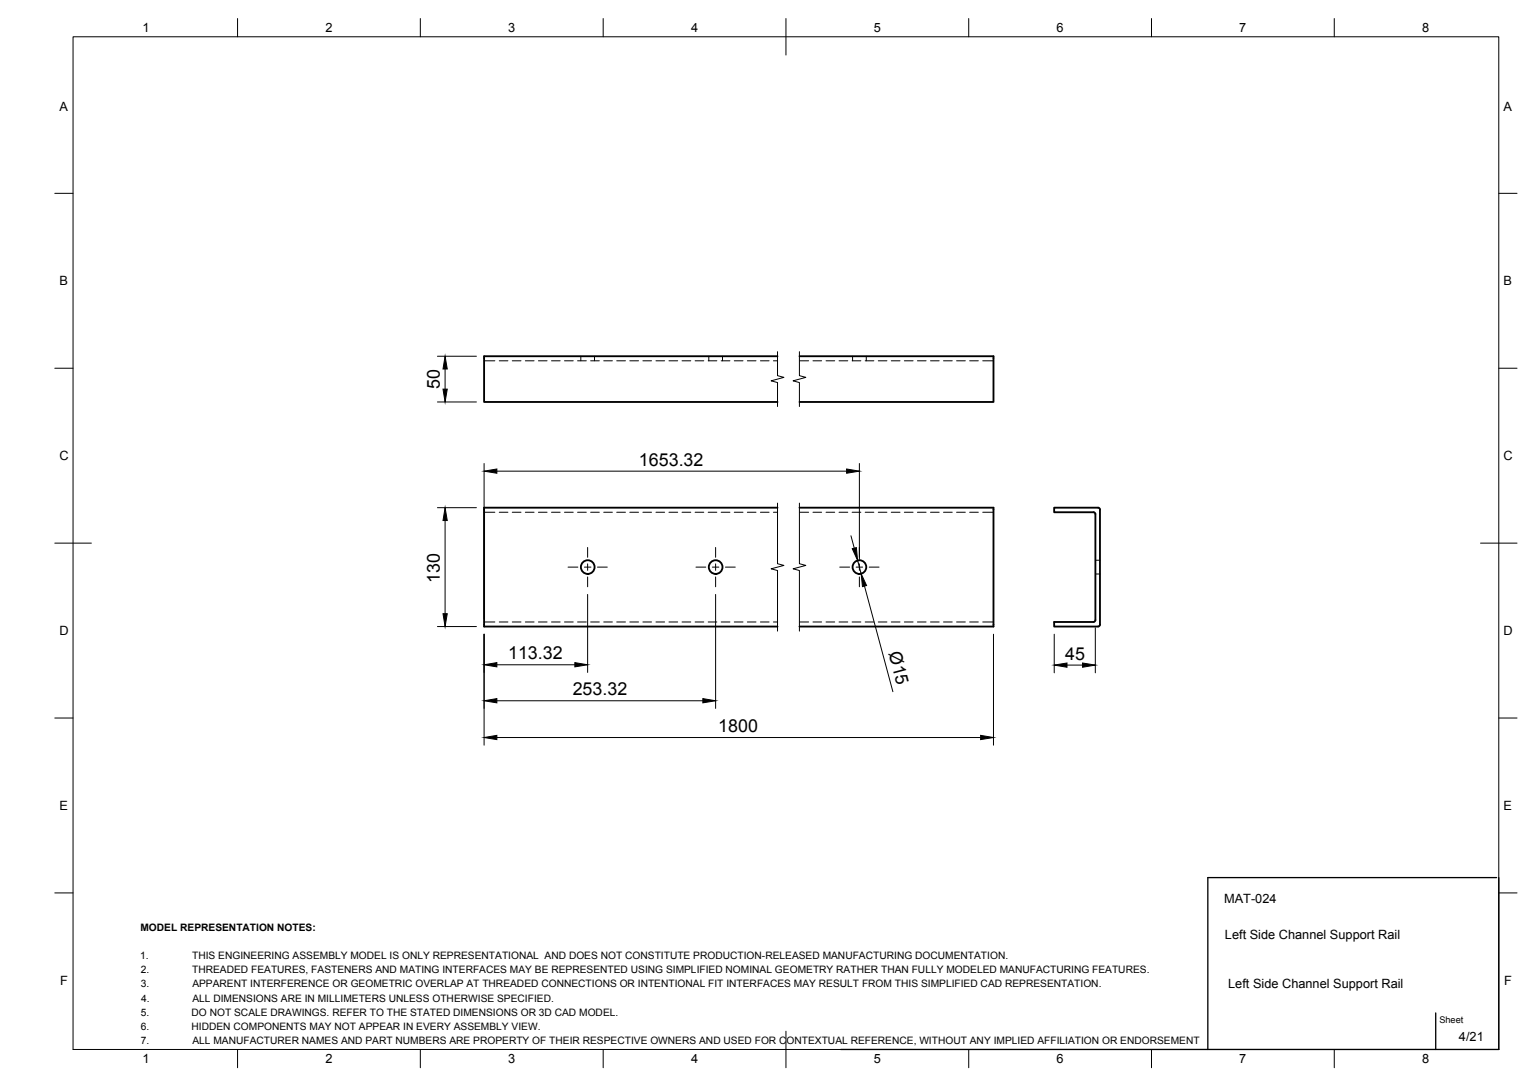
ISO-10303-21;
HEADER;
/* Generated by software containing ST-Developer
 * from STEP Tools, Inc. (www.steptools.com) 
 */

FILE_DESCRIPTION(
/* description */ ('STEP AP214'),
/* implementation_level */ '2;1');

FILE_NAME(
/* name */ 'Left Side Channel Support Rail.step',
/* time_stamp */ '2026-11-14T06:34:07-08:00',
/* author */ (''),
/* organization */ (''),
/* preprocessor_version */ 'ST-DEVELOPER v20.2',
/* originating_system */ 'Autodesk Translation Framework v15.17.0.0',
/* authorisation */ '');

FILE_SCHEMA (('AUTOMOTIVE_DESIGN { 1 0 10303 214 3 1 1 }'));
ENDSEC;

DATA;
#10=MECHANICAL_DESIGN_GEOMETRIC_PRESENTATION_REPRESENTATION('',(#7257),#310623);
#7223=SHAPE_REPRESENTATION_RELATIONSHIP('SRR','None',#310895,#7240);
#7240=ADVANCED_BREP_SHAPE_REPRESENTATION('',(#7325),#310604);
#7257=STYLED_ITEM('',(#311004),#7325);
#7325=MANIFOLD_SOLID_BREP('Body1',#93707);
#7415=FACE_BOUND('',#14492,.T.);
#7416=FACE_BOUND('',#14493,.T.);
#7417=FACE_BOUND('',#14494,.T.);
#7418=FACE_BOUND('',#14495,.T.);
#7419=FACE_BOUND('',#14496,.T.);
#7420=FACE_BOUND('',#14497,.T.);
#7421=FACE_BOUND('',#14498,.T.);
#7422=FACE_BOUND('',#14499,.T.);
#7423=FACE_BOUND('',#14500,.T.);
#7424=FACE_BOUND('',#14501,.T.);
#7425=FACE_BOUND('',#14502,.T.);
#7426=FACE_BOUND('',#14503,.T.);
#7427=FACE_BOUND('',#14508,.T.);
#7428=FACE_BOUND('',#14509,.T.);
#7429=FACE_BOUND('',#14510,.T.);
#7430=FACE_BOUND('',#14511,.T.);
#7431=FACE_BOUND('',#14512,.T.);
#7432=FACE_BOUND('',#14513,.T.);
#7433=FACE_BOUND('',#14514,.T.);
#7434=FACE_BOUND('',#14515,.T.);
#7435=FACE_BOUND('',#14516,.T.);
#7436=FACE_BOUND('',#14517,.T.);
#7437=FACE_BOUND('',#14518,.T.);
#7438=FACE_BOUND('',#14519,.T.);
#7716=PLANE('',#94060);
#7717=PLANE('',#94061);
#7718=PLANE('',#94062);
#7719=PLANE('',#94063);
#7720=PLANE('',#94064);
#7721=PLANE('',#94065);
#7722=PLANE('',#94066);
#7723=PLANE('',#94067);
#7724=PLANE('',#94068);
#7725=PLANE('',#94073);
#8714=FACE_OUTER_BOUND('',#14477,.T.);
#8715=FACE_OUTER_BOUND('',#14478,.T.);
#8716=FACE_OUTER_BOUND('',#14479,.T.);
#8717=FACE_OUTER_BOUND('',#14480,.T.);
#8718=FACE_OUTER_BOUND('',#14481,.T.);
#8719=FACE_OUTER_BOUND('',#14482,.T.);
#8720=FACE_OUTER_BOUND('',#14483,.T.);
#8721=FACE_OUTER_BOUND('',#14484,.T.);
#8722=FACE_OUTER_BOUND('',#14485,.T.);
#8723=FACE_OUTER_BOUND('',#14486,.T.);
#8724=FACE_OUTER_BOUND('',#14487,.T.);
#8725=FACE_OUTER_BOUND('',#14488,.T.);
#8726=FACE_OUTER_BOUND('',#14489,.T.);
#8727=FACE_OUTER_BOUND('',#14490,.T.);
#8728=FACE_OUTER_BOUND('',#14491,.T.);
#8729=FACE_OUTER_BOUND('',#14504,.T.);
#8730=FACE_OUTER_BOUND('',#14505,.T.);
#8731=FACE_OUTER_BOUND('',#14506,.T.);
#8732=FACE_OUTER_BOUND('',#14507,.T.);
#8733=FACE_OUTER_BOUND('',#14520,.T.);
#8734=FACE_OUTER_BOUND('',#14521,.T.);
#8735=FACE_OUTER_BOUND('',#14522,.T.);
#8736=FACE_OUTER_BOUND('',#14523,.T.);
#8737=FACE_OUTER_BOUND('',#14524,.T.);
#8738=FACE_OUTER_BOUND('',#14525,.T.);
#8739=FACE_OUTER_BOUND('',#14526,.T.);
#14477=EDGE_LOOP('',(#57801,#57802,#57803,#57804));
#14478=EDGE_LOOP('',(#57805,#57806,#57807,#57808));
#14479=EDGE_LOOP('',(#57809,#57810,#57811,#57812));
#14480=EDGE_LOOP('',(#57813,#57814,#57815,#57816));
#14481=EDGE_LOOP('',(#57817,#57818,#57819,#57820));
#14482=EDGE_LOOP('',(#57821,#57822,#57823,#57824));
#14483=EDGE_LOOP('',(#57825,#57826,#57827,#57828));
#14484=EDGE_LOOP('',(#57829,#57830,#57831,#57832));
#14485=EDGE_LOOP('',(#57833,#57834,#57835,#57836));
#14486=EDGE_LOOP('',(#57837,#57838,#57839,#57840));
#14487=EDGE_LOOP('',(#57841,#57842,#57843,#57844));
#14488=EDGE_LOOP('',(#57845,#57846,#57847,#57848));
#14489=EDGE_LOOP('',(#57849,#57850,#57851,#57852));
#14490=EDGE_LOOP('',(#57853,#57854,#57855,#57856));
#14491=EDGE_LOOP('',(#57857,#57858,#57859,#57860));
#14492=EDGE_LOOP('',(#57861));
#14493=EDGE_LOOP('',(#57862));
#14494=EDGE_LOOP('',(#57863));
#14495=EDGE_LOOP('',(#57864));
#14496=EDGE_LOOP('',(#57865));
#14497=EDGE_LOOP('',(#57866));
#14498=EDGE_LOOP('',(#57867));
#14499=EDGE_LOOP('',(#57868));
#14500=EDGE_LOOP('',(#57869));
#14501=EDGE_LOOP('',(#57870));
#14502=EDGE_LOOP('',(#57871));
#14503=EDGE_LOOP('',(#57872));
#14504=EDGE_LOOP('',(#57873,#57874,#57875,#57876));
#14505=EDGE_LOOP('',(#57877,#57878,#57879,#57880));
#14506=EDGE_LOOP('',(#57881,#57882,#57883,#57884));
#14507=EDGE_LOOP('',(#57885,#57886,#57887,#57888));
#14508=EDGE_LOOP('',(#57889));
#14509=EDGE_LOOP('',(#57890));
#14510=EDGE_LOOP('',(#57891));
#14511=EDGE_LOOP('',(#57892));
#14512=EDGE_LOOP('',(#57893));
#14513=EDGE_LOOP('',(#57894));
#14514=EDGE_LOOP('',(#57895));
#14515=EDGE_LOOP('',(#57896));
#14516=EDGE_LOOP('',(#57897));
#14517=EDGE_LOOP('',(#57898));
#14518=EDGE_LOOP('',(#57899));
#14519=EDGE_LOOP('',(#57900));
#14520=EDGE_LOOP('',(#57901,#57902,#57903,#57904));
#14521=EDGE_LOOP('',(#57905,#57906,#57907,#57908,#57909,#57910,#57911,#57912,
#57913,#57914,#57915,#57916));
#14522=EDGE_LOOP('',(#57917,#57918,#57919,#57920,#57921,#57922,#57923,#57924,
#57925,#57926,#57927,#57928));
#14523=EDGE_LOOP('',(#57929,#57930,#57931,#57932));
#14524=EDGE_LOOP('',(#57933,#57934,#57935,#57936));
#14525=EDGE_LOOP('',(#57937,#57938,#57939,#57940));
#14526=EDGE_LOOP('',(#57941,#57942,#57943,#57944));
#20521=LINE('',#131166,#24868);
#20522=LINE('',#131172,#24869);
#20523=LINE('',#131178,#24870);
#20524=LINE('',#131184,#24871);
#20525=LINE('',#131190,#24872);
#20526=LINE('',#131196,#24873);
#20527=LINE('',#131202,#24874);
#20528=LINE('',#131208,#24875);
#20529=LINE('',#131214,#24876);
#20530=LINE('',#131220,#24877);
#20531=LINE('',#131226,#24878);
#20532=LINE('',#131232,#24879);
#20533=LINE('',#131237,#24880);
#20534=LINE('',#131239,#24881);
#20535=LINE('',#131241,#24882);
#20536=LINE('',#131242,#24883);
#20537=LINE('',#131245,#24884);
#20538=LINE('',#131247,#24885);
#20539=LINE('',#131248,#24886);
#20540=LINE('',#131252,#24887);
#20541=LINE('',#131254,#24888);
#20542=LINE('',#131256,#24889);
#20543=LINE('',#131257,#24890);
#20544=LINE('',#131261,#24891);
#20545=LINE('',#131263,#24892);
#20546=LINE('',#131265,#24893);
#20547=LINE('',#131266,#24894);
#20548=LINE('',#131269,#24895);
#20549=LINE('',#131271,#24896);
#20550=LINE('',#131272,#24897);
#20551=LINE('',#131275,#24898);
#20552=LINE('',#131277,#24899);
#20553=LINE('',#131278,#24900);
#20554=LINE('',#131282,#24901);
#20555=LINE('',#131284,#24902);
#20556=LINE('',#131286,#24903);
#20557=LINE('',#131287,#24904);
#20558=LINE('',#131290,#24905);
#20559=LINE('',#131292,#24906);
#20560=LINE('',#131293,#24907);
#24868=VECTOR('',#105030,7.50000000000001);
#24869=VECTOR('',#105037,7.50000000000001);
#24870=VECTOR('',#105044,7.50000000000001);
#24871=VECTOR('',#105051,7.50000000000001);
#24872=VECTOR('',#105058,7.50000000000001);
#24873=VECTOR('',#105065,7.50000000000001);
#24874=VECTOR('',#105072,7.50000000000001);
#24875=VECTOR('',#105079,7.50000000000001);
#24876=VECTOR('',#105086,7.5);
#24877=VECTOR('',#105093,7.50000000000001);
#24878=VECTOR('',#105100,7.50000000000001);
#24879=VECTOR('',#105107,7.50000000000001);
#24880=VECTOR('',#105112,1000.);
#24881=VECTOR('',#105113,1000.);
#24882=VECTOR('',#105114,1000.);
#24883=VECTOR('',#105115,1000.);
#24884=VECTOR('',#105118,1000.);
#24885=VECTOR('',#105119,1000.);
#24886=VECTOR('',#105120,1000.);
#24887=VECTOR('',#105123,1000.);
#24888=VECTOR('',#105124,1000.);
#24889=VECTOR('',#105125,1000.);
#24890=VECTOR('',#105126,1000.);
#24891=VECTOR('',#105129,1000.);
#24892=VECTOR('',#105130,1000.);
#24893=VECTOR('',#105131,1000.);
#24894=VECTOR('',#105132,1000.);
#24895=VECTOR('',#105135,1000.);
#24896=VECTOR('',#105136,1000.);
#24897=VECTOR('',#105137,1000.);
#24898=VECTOR('',#105140,1000.);
#24899=VECTOR('',#105141,1000.);
#24900=VECTOR('',#105142,1000.);
#24901=VECTOR('',#105145,1000.);
#24902=VECTOR('',#105146,1000.);
#24903=VECTOR('',#105147,1000.);
#24904=VECTOR('',#105148,1000.);
#24905=VECTOR('',#105151,1000.);
#24906=VECTOR('',#105152,1000.);
#24907=VECTOR('',#105153,1000.);
#29207=CIRCLE('',#94025,7.50000000000001);
#29208=CIRCLE('',#94026,7.50000000000001);
#29209=CIRCLE('',#94028,7.50000000000001);
#29210=CIRCLE('',#94029,7.50000000000001);
#29211=CIRCLE('',#94031,7.50000000000001);
#29212=CIRCLE('',#94032,7.50000000000001);
#29213=CIRCLE('',#94034,7.50000000000001);
#29214=CIRCLE('',#94035,7.50000000000001);
#29215=CIRCLE('',#94037,7.50000000000001);
#29216=CIRCLE('',#94038,7.50000000000001);
#29217=CIRCLE('',#94040,7.50000000000001);
#29218=CIRCLE('',#94041,7.50000000000001);
#29219=CIRCLE('',#94043,7.50000000000001);
#29220=CIRCLE('',#94044,7.50000000000001);
#29221=CIRCLE('',#94046,7.50000000000001);
#29222=CIRCLE('',#94047,7.50000000000001);
#29223=CIRCLE('',#94049,7.5);
#29224=CIRCLE('',#94050,7.5);
#29225=CIRCLE('',#94052,7.50000000000001);
#29226=CIRCLE('',#94053,7.50000000000001);
#29227=CIRCLE('',#94055,7.50000000000001);
#29228=CIRCLE('',#94056,7.50000000000001);
#29229=CIRCLE('',#94058,7.50000000000001);
#29230=CIRCLE('',#94059,7.50000000000001);
#29231=CIRCLE('',#94069,2.);
#29232=CIRCLE('',#94070,2.);
#29233=CIRCLE('',#94071,2.);
#29234=CIRCLE('',#94072,2.);
#29235=CIRCLE('',#94074,2.);
#29236=CIRCLE('',#94075,2.);
#29237=CIRCLE('',#94076,2.);
#29238=CIRCLE('',#94077,2.);
#35153=VERTEX_POINT('',#131163);
#35154=VERTEX_POINT('',#131165);
#35155=VERTEX_POINT('',#131169);
#35156=VERTEX_POINT('',#131171);
#35157=VERTEX_POINT('',#131175);
#35158=VERTEX_POINT('',#131177);
#35159=VERTEX_POINT('',#131181);
#35160=VERTEX_POINT('',#131183);
#35161=VERTEX_POINT('',#131187);
#35162=VERTEX_POINT('',#131189);
#35163=VERTEX_POINT('',#131193);
#35164=VERTEX_POINT('',#131195);
#35165=VERTEX_POINT('',#131199);
#35166=VERTEX_POINT('',#131201);
#35167=VERTEX_POINT('',#131205);
#35168=VERTEX_POINT('',#131207);
#35169=VERTEX_POINT('',#131211);
#35170=VERTEX_POINT('',#131213);
#35171=VERTEX_POINT('',#131217);
#35172=VERTEX_POINT('',#131219);
#35173=VERTEX_POINT('',#131223);
#35174=VERTEX_POINT('',#131225);
#35175=VERTEX_POINT('',#131229);
#35176=VERTEX_POINT('',#131231);
#35177=VERTEX_POINT('',#131235);
#35178=VERTEX_POINT('',#131236);
#35179=VERTEX_POINT('',#131238);
#35180=VERTEX_POINT('',#131240);
#35181=VERTEX_POINT('',#131244);
#35182=VERTEX_POINT('',#131246);
#35183=VERTEX_POINT('',#131250);
#35184=VERTEX_POINT('',#131251);
#35185=VERTEX_POINT('',#131253);
#35186=VERTEX_POINT('',#131255);
#35187=VERTEX_POINT('',#131259);
#35188=VERTEX_POINT('',#131260);
#35189=VERTEX_POINT('',#131262);
#35190=VERTEX_POINT('',#131264);
#35191=VERTEX_POINT('',#131268);
#35192=VERTEX_POINT('',#131270);
#35193=VERTEX_POINT('',#131274);
#35194=VERTEX_POINT('',#131276);
#35195=VERTEX_POINT('',#131280);
#35196=VERTEX_POINT('',#131281);
#35197=VERTEX_POINT('',#131283);
#35198=VERTEX_POINT('',#131285);
#35199=VERTEX_POINT('',#131289);
#35200=VERTEX_POINT('',#131291);
#43680=EDGE_CURVE('',#35153,#35153,#29207,.T.);
#43681=EDGE_CURVE('',#35153,#35154,#20521,.T.);
#43682=EDGE_CURVE('',#35154,#35154,#29208,.T.);
#43683=EDGE_CURVE('',#35155,#35155,#29209,.T.);
#43684=EDGE_CURVE('',#35155,#35156,#20522,.T.);
#43685=EDGE_CURVE('',#35156,#35156,#29210,.T.);
#43686=EDGE_CURVE('',#35157,#35157,#29211,.T.);
#43687=EDGE_CURVE('',#35157,#35158,#20523,.T.);
#43688=EDGE_CURVE('',#35158,#35158,#29212,.T.);
#43689=EDGE_CURVE('',#35159,#35159,#29213,.T.);
#43690=EDGE_CURVE('',#35159,#35160,#20524,.T.);
#43691=EDGE_CURVE('',#35160,#35160,#29214,.T.);
#43692=EDGE_CURVE('',#35161,#35161,#29215,.T.);
#43693=EDGE_CURVE('',#35161,#35162,#20525,.T.);
#43694=EDGE_CURVE('',#35162,#35162,#29216,.T.);
#43695=EDGE_CURVE('',#35163,#35163,#29217,.T.);
#43696=EDGE_CURVE('',#35163,#35164,#20526,.T.);
#43697=EDGE_CURVE('',#35164,#35164,#29218,.T.);
#43698=EDGE_CURVE('',#35165,#35165,#29219,.T.);
#43699=EDGE_CURVE('',#35165,#35166,#20527,.T.);
#43700=EDGE_CURVE('',#35166,#35166,#29220,.T.);
#43701=EDGE_CURVE('',#35167,#35167,#29221,.T.);
#43702=EDGE_CURVE('',#35167,#35168,#20528,.T.);
#43703=EDGE_CURVE('',#35168,#35168,#29222,.T.);
#43704=EDGE_CURVE('',#35169,#35169,#29223,.T.);
#43705=EDGE_CURVE('',#35169,#35170,#20529,.T.);
#43706=EDGE_CURVE('',#35170,#35170,#29224,.T.);
#43707=EDGE_CURVE('',#35171,#35171,#29225,.T.);
#43708=EDGE_CURVE('',#35171,#35172,#20530,.T.);
#43709=EDGE_CURVE('',#35172,#35172,#29226,.T.);
#43710=EDGE_CURVE('',#35173,#35173,#29227,.T.);
#43711=EDGE_CURVE('',#35173,#35174,#20531,.T.);
#43712=EDGE_CURVE('',#35174,#35174,#29228,.T.);
#43713=EDGE_CURVE('',#35175,#35175,#29229,.T.);
#43714=EDGE_CURVE('',#35175,#35176,#20532,.T.);
#43715=EDGE_CURVE('',#35176,#35176,#29230,.T.);
#43716=EDGE_CURVE('',#35177,#35178,#20533,.T.);
#43717=EDGE_CURVE('',#35179,#35178,#20534,.T.);
#43718=EDGE_CURVE('',#35180,#35179,#20535,.T.);
#43719=EDGE_CURVE('',#35180,#35177,#20536,.T.);
#43720=EDGE_CURVE('',#35178,#35181,#20537,.T.);
#43721=EDGE_CURVE('',#35181,#35182,#20538,.T.);
#43722=EDGE_CURVE('',#35179,#35182,#20539,.T.);
#43723=EDGE_CURVE('',#35183,#35184,#20540,.T.);
#43724=EDGE_CURVE('',#35184,#35185,#20541,.T.);
#43725=EDGE_CURVE('',#35186,#35185,#20542,.T.);
#43726=EDGE_CURVE('',#35186,#35183,#20543,.T.);
#43727=EDGE_CURVE('',#35187,#35188,#20544,.T.);
#43728=EDGE_CURVE('',#35187,#35189,#20545,.T.);
#43729=EDGE_CURVE('',#35189,#35190,#20546,.T.);
#43730=EDGE_CURVE('',#35188,#35190,#20547,.T.);
#43731=EDGE_CURVE('',#35190,#35191,#20548,.T.);
#43732=EDGE_CURVE('',#35192,#35191,#20549,.T.);
#43733=EDGE_CURVE('',#35188,#35192,#20550,.T.);
#43734=EDGE_CURVE('',#35191,#35193,#20551,.T.);
#43735=EDGE_CURVE('',#35193,#35194,#20552,.T.);
#43736=EDGE_CURVE('',#35192,#35194,#20553,.T.);
#43737=EDGE_CURVE('',#35195,#35196,#20554,.T.);
#43738=EDGE_CURVE('',#35196,#35197,#20555,.T.);
#43739=EDGE_CURVE('',#35198,#35197,#20556,.T.);
#43740=EDGE_CURVE('',#35198,#35195,#20557,.T.);
#43741=EDGE_CURVE('',#35199,#35180,#20558,.T.);
#43742=EDGE_CURVE('',#35199,#35200,#20559,.T.);
#43743=EDGE_CURVE('',#35200,#35177,#20560,.T.);
#43744=EDGE_CURVE('',#35185,#35187,#29231,.T.);
#43745=EDGE_CURVE('',#35194,#35198,#29232,.T.);
#43746=EDGE_CURVE('',#35197,#35199,#29233,.T.);
#43747=EDGE_CURVE('',#35182,#35186,#29234,.T.);
#43748=EDGE_CURVE('',#35189,#35184,#29235,.T.);
#43749=EDGE_CURVE('',#35183,#35181,#29236,.T.);
#43750=EDGE_CURVE('',#35200,#35196,#29237,.T.);
#43751=EDGE_CURVE('',#35195,#35193,#29238,.T.);
#57801=ORIENTED_EDGE('',*,*,#43680,.F.);
#57802=ORIENTED_EDGE('',*,*,#43681,.T.);
#57803=ORIENTED_EDGE('',*,*,#43682,.T.);
#57804=ORIENTED_EDGE('',*,*,#43681,.F.);
#57805=ORIENTED_EDGE('',*,*,#43683,.F.);
#57806=ORIENTED_EDGE('',*,*,#43684,.T.);
#57807=ORIENTED_EDGE('',*,*,#43685,.T.);
#57808=ORIENTED_EDGE('',*,*,#43684,.F.);
#57809=ORIENTED_EDGE('',*,*,#43686,.F.);
#57810=ORIENTED_EDGE('',*,*,#43687,.T.);
#57811=ORIENTED_EDGE('',*,*,#43688,.T.);
#57812=ORIENTED_EDGE('',*,*,#43687,.F.);
#57813=ORIENTED_EDGE('',*,*,#43689,.F.);
#57814=ORIENTED_EDGE('',*,*,#43690,.T.);
#57815=ORIENTED_EDGE('',*,*,#43691,.T.);
#57816=ORIENTED_EDGE('',*,*,#43690,.F.);
#57817=ORIENTED_EDGE('',*,*,#43692,.F.);
#57818=ORIENTED_EDGE('',*,*,#43693,.T.);
#57819=ORIENTED_EDGE('',*,*,#43694,.T.);
#57820=ORIENTED_EDGE('',*,*,#43693,.F.);
#57821=ORIENTED_EDGE('',*,*,#43695,.F.);
#57822=ORIENTED_EDGE('',*,*,#43696,.T.);
#57823=ORIENTED_EDGE('',*,*,#43697,.T.);
#57824=ORIENTED_EDGE('',*,*,#43696,.F.);
#57825=ORIENTED_EDGE('',*,*,#43698,.F.);
#57826=ORIENTED_EDGE('',*,*,#43699,.T.);
#57827=ORIENTED_EDGE('',*,*,#43700,.T.);
#57828=ORIENTED_EDGE('',*,*,#43699,.F.);
#57829=ORIENTED_EDGE('',*,*,#43701,.F.);
#57830=ORIENTED_EDGE('',*,*,#43702,.T.);
#57831=ORIENTED_EDGE('',*,*,#43703,.T.);
#57832=ORIENTED_EDGE('',*,*,#43702,.F.);
#57833=ORIENTED_EDGE('',*,*,#43704,.F.);
#57834=ORIENTED_EDGE('',*,*,#43705,.T.);
#57835=ORIENTED_EDGE('',*,*,#43706,.T.);
#57836=ORIENTED_EDGE('',*,*,#43705,.F.);
#57837=ORIENTED_EDGE('',*,*,#43707,.F.);
#57838=ORIENTED_EDGE('',*,*,#43708,.T.);
#57839=ORIENTED_EDGE('',*,*,#43709,.T.);
#57840=ORIENTED_EDGE('',*,*,#43708,.F.);
#57841=ORIENTED_EDGE('',*,*,#43710,.F.);
#57842=ORIENTED_EDGE('',*,*,#43711,.T.);
#57843=ORIENTED_EDGE('',*,*,#43712,.T.);
#57844=ORIENTED_EDGE('',*,*,#43711,.F.);
#57845=ORIENTED_EDGE('',*,*,#43713,.F.);
#57846=ORIENTED_EDGE('',*,*,#43714,.T.);
#57847=ORIENTED_EDGE('',*,*,#43715,.T.);
#57848=ORIENTED_EDGE('',*,*,#43714,.F.);
#57849=ORIENTED_EDGE('',*,*,#43716,.T.);
#57850=ORIENTED_EDGE('',*,*,#43717,.F.);
#57851=ORIENTED_EDGE('',*,*,#43718,.F.);
#57852=ORIENTED_EDGE('',*,*,#43719,.T.);
#57853=ORIENTED_EDGE('',*,*,#43720,.T.);
#57854=ORIENTED_EDGE('',*,*,#43721,.T.);
#57855=ORIENTED_EDGE('',*,*,#43722,.F.);
#57856=ORIENTED_EDGE('',*,*,#43717,.T.);
#57857=ORIENTED_EDGE('',*,*,#43723,.T.);
#57858=ORIENTED_EDGE('',*,*,#43724,.T.);
#57859=ORIENTED_EDGE('',*,*,#43725,.F.);
#57860=ORIENTED_EDGE('',*,*,#43726,.T.);
#57861=ORIENTED_EDGE('',*,*,#43680,.T.);
#57862=ORIENTED_EDGE('',*,*,#43683,.T.);
#57863=ORIENTED_EDGE('',*,*,#43686,.T.);
#57864=ORIENTED_EDGE('',*,*,#43689,.T.);
#57865=ORIENTED_EDGE('',*,*,#43692,.T.);
#57866=ORIENTED_EDGE('',*,*,#43695,.T.);
#57867=ORIENTED_EDGE('',*,*,#43698,.T.);
#57868=ORIENTED_EDGE('',*,*,#43701,.T.);
#57869=ORIENTED_EDGE('',*,*,#43704,.T.);
#57870=ORIENTED_EDGE('',*,*,#43707,.T.);
#57871=ORIENTED_EDGE('',*,*,#43710,.T.);
#57872=ORIENTED_EDGE('',*,*,#43713,.T.);
#57873=ORIENTED_EDGE('',*,*,#43727,.F.);
#57874=ORIENTED_EDGE('',*,*,#43728,.T.);
#57875=ORIENTED_EDGE('',*,*,#43729,.T.);
#57876=ORIENTED_EDGE('',*,*,#43730,.F.);
#57877=ORIENTED_EDGE('',*,*,#43731,.T.);
#57878=ORIENTED_EDGE('',*,*,#43732,.F.);
#57879=ORIENTED_EDGE('',*,*,#43733,.F.);
#57880=ORIENTED_EDGE('',*,*,#43730,.T.);
#57881=ORIENTED_EDGE('',*,*,#43734,.T.);
#57882=ORIENTED_EDGE('',*,*,#43735,.T.);
#57883=ORIENTED_EDGE('',*,*,#43736,.F.);
#57884=ORIENTED_EDGE('',*,*,#43732,.T.);
#57885=ORIENTED_EDGE('',*,*,#43737,.T.);
#57886=ORIENTED_EDGE('',*,*,#43738,.T.);
#57887=ORIENTED_EDGE('',*,*,#43739,.F.);
#57888=ORIENTED_EDGE('',*,*,#43740,.T.);
#57889=ORIENTED_EDGE('',*,*,#43682,.F.);
#57890=ORIENTED_EDGE('',*,*,#43685,.F.);
#57891=ORIENTED_EDGE('',*,*,#43688,.F.);
#57892=ORIENTED_EDGE('',*,*,#43691,.F.);
#57893=ORIENTED_EDGE('',*,*,#43694,.F.);
#57894=ORIENTED_EDGE('',*,*,#43697,.F.);
#57895=ORIENTED_EDGE('',*,*,#43700,.F.);
#57896=ORIENTED_EDGE('',*,*,#43703,.F.);
#57897=ORIENTED_EDGE('',*,*,#43706,.F.);
#57898=ORIENTED_EDGE('',*,*,#43709,.F.);
#57899=ORIENTED_EDGE('',*,*,#43712,.F.);
#57900=ORIENTED_EDGE('',*,*,#43715,.F.);
#57901=ORIENTED_EDGE('',*,*,#43741,.F.);
#57902=ORIENTED_EDGE('',*,*,#43742,.T.);
#57903=ORIENTED_EDGE('',*,*,#43743,.T.);
#57904=ORIENTED_EDGE('',*,*,#43719,.F.);
#57905=ORIENTED_EDGE('',*,*,#43725,.T.);
#57906=ORIENTED_EDGE('',*,*,#43744,.T.);
#57907=ORIENTED_EDGE('',*,*,#43727,.T.);
#57908=ORIENTED_EDGE('',*,*,#43733,.T.);
#57909=ORIENTED_EDGE('',*,*,#43736,.T.);
#57910=ORIENTED_EDGE('',*,*,#43745,.T.);
#57911=ORIENTED_EDGE('',*,*,#43739,.T.);
#57912=ORIENTED_EDGE('',*,*,#43746,.T.);
#57913=ORIENTED_EDGE('',*,*,#43741,.T.);
#57914=ORIENTED_EDGE('',*,*,#43718,.T.);
#57915=ORIENTED_EDGE('',*,*,#43722,.T.);
#57916=ORIENTED_EDGE('',*,*,#43747,.T.);
#57917=ORIENTED_EDGE('',*,*,#43729,.F.);
#57918=ORIENTED_EDGE('',*,*,#43748,.T.);
#57919=ORIENTED_EDGE('',*,*,#43723,.F.);
#57920=ORIENTED_EDGE('',*,*,#43749,.T.);
#57921=ORIENTED_EDGE('',*,*,#43720,.F.);
#57922=ORIENTED_EDGE('',*,*,#43716,.F.);
#57923=ORIENTED_EDGE('',*,*,#43743,.F.);
#57924=ORIENTED_EDGE('',*,*,#43750,.T.);
#57925=ORIENTED_EDGE('',*,*,#43737,.F.);
#57926=ORIENTED_EDGE('',*,*,#43751,.T.);
#57927=ORIENTED_EDGE('',*,*,#43734,.F.);
#57928=ORIENTED_EDGE('',*,*,#43731,.F.);
#57929=ORIENTED_EDGE('',*,*,#43744,.F.);
#57930=ORIENTED_EDGE('',*,*,#43724,.F.);
#57931=ORIENTED_EDGE('',*,*,#43748,.F.);
#57932=ORIENTED_EDGE('',*,*,#43728,.F.);
#57933=ORIENTED_EDGE('',*,*,#43747,.F.);
#57934=ORIENTED_EDGE('',*,*,#43721,.F.);
#57935=ORIENTED_EDGE('',*,*,#43749,.F.);
#57936=ORIENTED_EDGE('',*,*,#43726,.F.);
#57937=ORIENTED_EDGE('',*,*,#43746,.F.);
#57938=ORIENTED_EDGE('',*,*,#43738,.F.);
#57939=ORIENTED_EDGE('',*,*,#43750,.F.);
#57940=ORIENTED_EDGE('',*,*,#43742,.F.);
#57941=ORIENTED_EDGE('',*,*,#43745,.F.);
#57942=ORIENTED_EDGE('',*,*,#43735,.F.);
#57943=ORIENTED_EDGE('',*,*,#43751,.F.);
#57944=ORIENTED_EDGE('',*,*,#43740,.F.);
#85771=CYLINDRICAL_SURFACE('',#94024,7.50000000000001);
#85772=CYLINDRICAL_SURFACE('',#94027,7.50000000000001);
#85773=CYLINDRICAL_SURFACE('',#94030,7.50000000000001);
#85774=CYLINDRICAL_SURFACE('',#94033,7.50000000000001);
#85775=CYLINDRICAL_SURFACE('',#94036,7.50000000000001);
#85776=CYLINDRICAL_SURFACE('',#94039,7.50000000000001);
#85777=CYLINDRICAL_SURFACE('',#94042,7.50000000000001);
#85778=CYLINDRICAL_SURFACE('',#94045,7.50000000000001);
#85779=CYLINDRICAL_SURFACE('',#94048,7.5);
#85780=CYLINDRICAL_SURFACE('',#94051,7.50000000000001);
#85781=CYLINDRICAL_SURFACE('',#94054,7.50000000000001);
#85782=CYLINDRICAL_SURFACE('',#94057,7.50000000000001);
#85783=CYLINDRICAL_SURFACE('',#94078,2.);
#85784=CYLINDRICAL_SURFACE('',#94079,2.);
#85785=CYLINDRICAL_SURFACE('',#94080,2.);
#85786=CYLINDRICAL_SURFACE('',#94081,2.);
#87993=ADVANCED_FACE('',(#8714),#85771,.F.);
#87994=ADVANCED_FACE('',(#8715),#85772,.F.);
#87995=ADVANCED_FACE('',(#8716),#85773,.F.);
#87996=ADVANCED_FACE('',(#8717),#85774,.F.);
#87997=ADVANCED_FACE('',(#8718),#85775,.F.);
#87998=ADVANCED_FACE('',(#8719),#85776,.F.);
#87999=ADVANCED_FACE('',(#8720),#85777,.F.);
#88000=ADVANCED_FACE('',(#8721),#85778,.F.);
#88001=ADVANCED_FACE('',(#8722),#85779,.F.);
#88002=ADVANCED_FACE('',(#8723),#85780,.F.);
#88003=ADVANCED_FACE('',(#8724),#85781,.F.);
#88004=ADVANCED_FACE('',(#8725),#85782,.F.);
#88005=ADVANCED_FACE('',(#8726),#7716,.F.);
#88006=ADVANCED_FACE('',(#8727),#7717,.F.);
#88007=ADVANCED_FACE('',(#8728,#7415,#7416,#7417,#7418,#7419,#7420,#7421,
#7422,#7423,#7424,#7425,#7426),#7718,.F.);
#88008=ADVANCED_FACE('',(#8729),#7719,.F.);
#88009=ADVANCED_FACE('',(#8730),#7720,.F.);
#88010=ADVANCED_FACE('',(#8731),#7721,.F.);
#88011=ADVANCED_FACE('',(#8732,#7427,#7428,#7429,#7430,#7431,#7432,#7433,
#7434,#7435,#7436,#7437,#7438),#7722,.F.);
#88012=ADVANCED_FACE('',(#8733),#7723,.F.);
#88013=ADVANCED_FACE('',(#8734),#7724,.T.);
#88014=ADVANCED_FACE('',(#8735),#7725,.F.);
#88015=ADVANCED_FACE('',(#8736),#85783,.T.);
#88016=ADVANCED_FACE('',(#8737),#85784,.T.);
#88017=ADVANCED_FACE('',(#8738),#85785,.F.);
#88018=ADVANCED_FACE('',(#8739),#85786,.F.);
#93707=CLOSED_SHELL('',(#87993,#87994,#87995,#87996,#87997,#87998,#87999,
#88000,#88001,#88002,#88003,#88004,#88005,#88006,#88007,#88008,#88009,#88010,
#88011,#88012,#88013,#88014,#88015,#88016,#88017,#88018));
#94023=AXIS2_PLACEMENT_3D('',#131161,#105024,#105025);
#94024=AXIS2_PLACEMENT_3D('',#131162,#105026,#105027);
#94025=AXIS2_PLACEMENT_3D('',#131164,#105028,#105029);
#94026=AXIS2_PLACEMENT_3D('',#131167,#105031,#105032);
#94027=AXIS2_PLACEMENT_3D('',#131168,#105033,#105034);
#94028=AXIS2_PLACEMENT_3D('',#131170,#105035,#105036);
#94029=AXIS2_PLACEMENT_3D('',#131173,#105038,#105039);
#94030=AXIS2_PLACEMENT_3D('',#131174,#105040,#105041);
#94031=AXIS2_PLACEMENT_3D('',#131176,#105042,#105043);
#94032=AXIS2_PLACEMENT_3D('',#131179,#105045,#105046);
#94033=AXIS2_PLACEMENT_3D('',#131180,#105047,#105048);
#94034=AXIS2_PLACEMENT_3D('',#131182,#105049,#105050);
#94035=AXIS2_PLACEMENT_3D('',#131185,#105052,#105053);
#94036=AXIS2_PLACEMENT_3D('',#131186,#105054,#105055);
#94037=AXIS2_PLACEMENT_3D('',#131188,#105056,#105057);
#94038=AXIS2_PLACEMENT_3D('',#131191,#105059,#105060);
#94039=AXIS2_PLACEMENT_3D('',#131192,#105061,#105062);
#94040=AXIS2_PLACEMENT_3D('',#131194,#105063,#105064);
#94041=AXIS2_PLACEMENT_3D('',#131197,#105066,#105067);
#94042=AXIS2_PLACEMENT_3D('',#131198,#105068,#105069);
#94043=AXIS2_PLACEMENT_3D('',#131200,#105070,#105071);
#94044=AXIS2_PLACEMENT_3D('',#131203,#105073,#105074);
#94045=AXIS2_PLACEMENT_3D('',#131204,#105075,#105076);
#94046=AXIS2_PLACEMENT_3D('',#131206,#105077,#105078);
#94047=AXIS2_PLACEMENT_3D('',#131209,#105080,#105081);
#94048=AXIS2_PLACEMENT_3D('',#131210,#105082,#105083);
#94049=AXIS2_PLACEMENT_3D('',#131212,#105084,#105085);
#94050=AXIS2_PLACEMENT_3D('',#131215,#105087,#105088);
#94051=AXIS2_PLACEMENT_3D('',#131216,#105089,#105090);
#94052=AXIS2_PLACEMENT_3D('',#131218,#105091,#105092);
#94053=AXIS2_PLACEMENT_3D('',#131221,#105094,#105095);
#94054=AXIS2_PLACEMENT_3D('',#131222,#105096,#105097);
#94055=AXIS2_PLACEMENT_3D('',#131224,#105098,#105099);
#94056=AXIS2_PLACEMENT_3D('',#131227,#105101,#105102);
#94057=AXIS2_PLACEMENT_3D('',#131228,#105103,#105104);
#94058=AXIS2_PLACEMENT_3D('',#131230,#105105,#105106);
#94059=AXIS2_PLACEMENT_3D('',#131233,#105108,#105109);
#94060=AXIS2_PLACEMENT_3D('',#131234,#105110,#105111);
#94061=AXIS2_PLACEMENT_3D('',#131243,#105116,#105117);
#94062=AXIS2_PLACEMENT_3D('',#131249,#105121,#105122);
#94063=AXIS2_PLACEMENT_3D('',#131258,#105127,#105128);
#94064=AXIS2_PLACEMENT_3D('',#131267,#105133,#105134);
#94065=AXIS2_PLACEMENT_3D('',#131273,#105138,#105139);
#94066=AXIS2_PLACEMENT_3D('',#131279,#105143,#105144);
#94067=AXIS2_PLACEMENT_3D('',#131288,#105149,#105150);
#94068=AXIS2_PLACEMENT_3D('',#131294,#105154,#105155);
#94069=AXIS2_PLACEMENT_3D('',#131295,#105156,#105157);
#94070=AXIS2_PLACEMENT_3D('',#131296,#105158,#105159);
#94071=AXIS2_PLACEMENT_3D('',#131297,#105160,#105161);
#94072=AXIS2_PLACEMENT_3D('',#131298,#105162,#105163);
#94073=AXIS2_PLACEMENT_3D('',#131299,#105164,#105165);
#94074=AXIS2_PLACEMENT_3D('',#131300,#105166,#105167);
#94075=AXIS2_PLACEMENT_3D('',#131301,#105168,#105169);
#94076=AXIS2_PLACEMENT_3D('',#131302,#105170,#105171);
#94077=AXIS2_PLACEMENT_3D('',#131303,#105172,#105173);
#94078=AXIS2_PLACEMENT_3D('',#131304,#105174,#105175);
#94079=AXIS2_PLACEMENT_3D('',#131305,#105176,#105177);
#94080=AXIS2_PLACEMENT_3D('',#131306,#105178,#105179);
#94081=AXIS2_PLACEMENT_3D('',#131307,#105180,#105181);
#105024=DIRECTION('axis',(0.,0.,1.));
#105025=DIRECTION('refdir',(1.,0.,0.));
#105026=DIRECTION('center_axis',(1.,0.,-2.89120579329468E-17));
#105027=DIRECTION('ref_axis',(-2.89120579329468E-17,0.,-1.));
#105028=DIRECTION('center_axis',(1.,0.,-5.33761069531325E-17));
#105029=DIRECTION('ref_axis',(-5.33761069531325E-17,0.,-1.));
#105030=DIRECTION('',(1.,0.,-2.89120579329468E-17));
#105031=DIRECTION('center_axis',(1.,0.,-2.96720509643778E-17));
#105032=DIRECTION('ref_axis',(-2.96720509643778E-17,0.,-1.));
#105033=DIRECTION('center_axis',(1.,0.,-2.89120579329468E-17));
#105034=DIRECTION('ref_axis',(-2.89120579329468E-17,0.,-1.));
#105035=DIRECTION('center_axis',(1.,0.,-5.33761069531325E-17));
#105036=DIRECTION('ref_axis',(-5.33761069531325E-17,0.,-1.));
#105037=DIRECTION('',(1.,0.,-2.89120579329468E-17));
#105038=DIRECTION('center_axis',(1.,0.,-2.89120579329468E-17));
#105039=DIRECTION('ref_axis',(-2.89120579329468E-17,0.,-1.));
#105040=DIRECTION('center_axis',(1.,0.,-2.89120579329468E-17));
#105041=DIRECTION('ref_axis',(-2.89120579329468E-17,0.,-1.));
#105042=DIRECTION('center_axis',(1.,0.,-5.33761069531325E-17));
#105043=DIRECTION('ref_axis',(-5.33761069531325E-17,0.,-1.));
#105044=DIRECTION('',(1.,0.,-2.89120579329468E-17));
#105045=DIRECTION('center_axis',(1.,0.,-2.89120579329468E-17));
#105046=DIRECTION('ref_axis',(-2.89120579329468E-17,0.,-1.));
#105047=DIRECTION('center_axis',(1.,0.,-2.89120579329468E-17));
#105048=DIRECTION('ref_axis',(-2.89120579329468E-17,0.,-1.));
#105049=DIRECTION('center_axis',(1.,0.,-5.33761069531325E-17));
#105050=DIRECTION('ref_axis',(-5.33761069531325E-17,0.,-1.));
#105051=DIRECTION('',(1.,0.,-2.89120579329468E-17));
#105052=DIRECTION('center_axis',(1.,0.,-2.96720509643778E-17));
#105053=DIRECTION('ref_axis',(-2.96720509643778E-17,0.,-1.));
#105054=DIRECTION('center_axis',(1.,0.,-2.89120579329468E-17));
#105055=DIRECTION('ref_axis',(-2.89120579329468E-17,0.,-1.));
#105056=DIRECTION('center_axis',(1.,0.,-5.33761069531325E-17));
#105057=DIRECTION('ref_axis',(-5.33761069531325E-17,0.,-1.));
#105058=DIRECTION('',(1.,0.,-2.89120579329468E-17));
#105059=DIRECTION('center_axis',(1.,0.,-2.96720509643778E-17));
#105060=DIRECTION('ref_axis',(-2.96720509643778E-17,0.,-1.));
#105061=DIRECTION('center_axis',(1.,0.,-2.89120579329468E-17));
#105062=DIRECTION('ref_axis',(-2.89120579329468E-17,0.,-1.));
#105063=DIRECTION('center_axis',(1.,0.,-5.33761069531325E-17));
#105064=DIRECTION('ref_axis',(-5.33761069531325E-17,0.,-1.));
#105065=DIRECTION('',(1.,0.,-2.89120579329468E-17));
#105066=DIRECTION('center_axis',(1.,0.,-2.96720509643778E-17));
#105067=DIRECTION('ref_axis',(-2.96720509643778E-17,0.,-1.));
#105068=DIRECTION('center_axis',(1.,0.,-2.89120579329468E-17));
#105069=DIRECTION('ref_axis',(-2.89120579329468E-17,0.,-1.));
#105070=DIRECTION('center_axis',(1.,0.,-5.33761069531325E-17));
#105071=DIRECTION('ref_axis',(-5.33761069531325E-17,0.,-1.));
#105072=DIRECTION('',(1.,0.,-2.89120579329468E-17));
#105073=DIRECTION('center_axis',(1.,0.,-2.96720509643778E-17));
#105074=DIRECTION('ref_axis',(-2.96720509643778E-17,0.,-1.));
#105075=DIRECTION('center_axis',(1.,0.,-2.89120579329468E-17));
#105076=DIRECTION('ref_axis',(-2.89120579329468E-17,0.,-1.));
#105077=DIRECTION('center_axis',(1.,0.,-5.33761069531325E-17));
#105078=DIRECTION('ref_axis',(-5.33761069531325E-17,0.,-1.));
#105079=DIRECTION('',(1.,0.,-2.89120579329468E-17));
#105080=DIRECTION('center_axis',(1.,0.,-2.96720509643778E-17));
#105081=DIRECTION('ref_axis',(-2.96720509643778E-17,0.,-1.));
#105082=DIRECTION('center_axis',(1.,0.,-2.89120579329468E-17));
#105083=DIRECTION('ref_axis',(-2.89120579329468E-17,0.,-1.));
#105084=DIRECTION('center_axis',(1.,0.,-5.33761069531325E-17));
#105085=DIRECTION('ref_axis',(-5.33761069531325E-17,0.,-1.));
#105086=DIRECTION('',(1.,0.,-2.89120579329468E-17));
#105087=DIRECTION('center_axis',(1.,0.,-2.96720509643778E-17));
#105088=DIRECTION('ref_axis',(-2.96720509643778E-17,0.,-1.));
#105089=DIRECTION('center_axis',(1.,0.,-2.89120579329468E-17));
#105090=DIRECTION('ref_axis',(-2.89120579329468E-17,0.,-1.));
#105091=DIRECTION('center_axis',(1.,0.,-5.33761069531325E-17));
#105092=DIRECTION('ref_axis',(-5.33761069531325E-17,0.,-1.));
#105093=DIRECTION('',(1.,0.,-2.89120579329468E-17));
#105094=DIRECTION('center_axis',(1.,0.,-2.96720509643778E-17));
#105095=DIRECTION('ref_axis',(-2.96720509643778E-17,0.,-1.));
#105096=DIRECTION('center_axis',(1.,0.,-2.89120579329468E-17));
#105097=DIRECTION('ref_axis',(-2.89120579329468E-17,0.,-1.));
#105098=DIRECTION('center_axis',(1.,0.,-5.33761069531325E-17));
#105099=DIRECTION('ref_axis',(-5.33761069531325E-17,0.,-1.));
#105100=DIRECTION('',(1.,0.,-2.89120579329468E-17));
#105101=DIRECTION('center_axis',(1.,0.,-2.96720509643778E-17));
#105102=DIRECTION('ref_axis',(-2.96720509643778E-17,0.,-1.));
#105103=DIRECTION('center_axis',(1.,0.,-2.89120579329468E-17));
#105104=DIRECTION('ref_axis',(-2.89120579329468E-17,0.,-1.));
#105105=DIRECTION('center_axis',(1.,0.,-5.33761069531325E-17));
#105106=DIRECTION('ref_axis',(-5.33761069531325E-17,0.,-1.));
#105107=DIRECTION('',(1.,0.,-2.89120579329468E-17));
#105108=DIRECTION('center_axis',(1.,0.,-2.96720509643778E-17));
#105109=DIRECTION('ref_axis',(-2.96720509643778E-17,0.,-1.));
#105110=DIRECTION('center_axis',(-1.,0.,0.));
#105111=DIRECTION('ref_axis',(0.,0.,1.));
#105112=DIRECTION('',(0.,0.,-1.));
#105113=DIRECTION('',(0.,-1.,0.));
#105114=DIRECTION('',(0.,0.,-1.));
#105115=DIRECTION('',(0.,-1.,0.));
#105116=DIRECTION('center_axis',(1.22464679914735E-16,0.,1.));
#105117=DIRECTION('ref_axis',(1.,0.,-1.22464679914735E-16));
#105118=DIRECTION('',(-1.,0.,1.22464679914735E-16));
#105119=DIRECTION('',(0.,1.,0.));
#105120=DIRECTION('',(-1.,0.,1.22464679914735E-16));
#105121=DIRECTION('center_axis',(1.,0.,-5.33761069531325E-17));
#105122=DIRECTION('ref_axis',(-5.33761069531325E-17,0.,-1.));
#105123=DIRECTION('',(5.33761069531325E-17,0.,1.));
#105124=DIRECTION('',(0.,1.,0.));
#105125=DIRECTION('',(5.33761069531325E-17,0.,1.));
#105126=DIRECTION('',(0.,-1.,0.));
#105127=DIRECTION('center_axis',(0.,0.,-1.));
#105128=DIRECTION('ref_axis',(-1.,0.,0.));
#105129=DIRECTION('',(1.,0.,0.));
#105130=DIRECTION('',(0.,-1.,0.));
#105131=DIRECTION('',(1.,0.,0.));
#105132=DIRECTION('',(0.,-1.,0.));
#105133=DIRECTION('center_axis',(-1.,0.,0.));
#105134=DIRECTION('ref_axis',(0.,0.,1.));
#105135=DIRECTION('',(0.,0.,-1.));
#105136=DIRECTION('',(0.,-1.,0.));
#105137=DIRECTION('',(0.,0.,-1.));
#105138=DIRECTION('center_axis',(0.,0.,1.));
#105139=DIRECTION('ref_axis',(1.,0.,0.));
#105140=DIRECTION('',(-1.,0.,0.));
#105141=DIRECTION('',(0.,1.,0.));
#105142=DIRECTION('',(-1.,0.,0.));
#105143=DIRECTION('center_axis',(-1.,0.,5.78241158658936E-17));
#105144=DIRECTION('ref_axis',(5.78241158658936E-17,0.,1.));
#105145=DIRECTION('',(-5.78241158658936E-17,0.,-1.));
#105146=DIRECTION('',(0.,1.,0.));
#105147=DIRECTION('',(-5.78241158658936E-17,0.,-1.));
#105148=DIRECTION('',(0.,-1.,0.));
#105149=DIRECTION('center_axis',(-7.70988211545248E-17,0.,-1.));
#105150=DIRECTION('ref_axis',(-1.,0.,7.70988211545248E-17));
#105151=DIRECTION('',(1.,0.,-7.70988211545248E-17));
#105152=DIRECTION('',(0.,-1.,0.));
#105153=DIRECTION('',(1.,0.,-7.70988211545248E-17));
#105154=DIRECTION('center_axis',(0.,1.,0.));
#105155=DIRECTION('ref_axis',(0.,0.,1.));
#105156=DIRECTION('center_axis',(0.,1.,0.));
#105157=DIRECTION('ref_axis',(0.,0.,1.));
#105158=DIRECTION('center_axis',(0.,-1.,0.));
#105159=DIRECTION('ref_axis',(0.,0.,1.));
#105160=DIRECTION('center_axis',(0.,-1.,0.));
#105161=DIRECTION('ref_axis',(0.,0.,1.));
#105162=DIRECTION('center_axis',(0.,1.,0.));
#105163=DIRECTION('ref_axis',(0.,0.,1.));
#105164=DIRECTION('center_axis',(0.,1.,0.));
#105165=DIRECTION('ref_axis',(0.,0.,1.));
#105166=DIRECTION('center_axis',(0.,-1.,0.));
#105167=DIRECTION('ref_axis',(0.,0.,1.));
#105168=DIRECTION('center_axis',(0.,-1.,0.));
#105169=DIRECTION('ref_axis',(0.,0.,1.));
#105170=DIRECTION('center_axis',(0.,1.,0.));
#105171=DIRECTION('ref_axis',(0.,0.,1.));
#105172=DIRECTION('center_axis',(0.,1.,0.));
#105173=DIRECTION('ref_axis',(0.,0.,1.));
#105174=DIRECTION('center_axis',(0.,-1.,0.));
#105175=DIRECTION('ref_axis',(0.,0.,-1.));
#105176=DIRECTION('center_axis',(0.,-1.,0.));
#105177=DIRECTION('ref_axis',(0.,0.,-1.));
#105178=DIRECTION('center_axis',(0.,1.,0.));
#105179=DIRECTION('ref_axis',(0.,0.,1.));
#105180=DIRECTION('center_axis',(0.,1.,0.));
#105181=DIRECTION('ref_axis',(0.,0.,1.));
#131161=CARTESIAN_POINT('',(0.,0.,0.));
#131162=CARTESIAN_POINT('Origin',(-55.,-753.32045741381,64.9999999999994));
#131163=CARTESIAN_POINT('',(-50.,-753.32045741381,72.4999999999994));
#131164=CARTESIAN_POINT('Origin',(-50.,-753.32045741381,64.9999999999994));
#131165=CARTESIAN_POINT('',(-45.,-753.32045741381,72.4999999999994));
#131166=CARTESIAN_POINT('',(-55.,-753.32045741381,72.4999999999994));
#131167=CARTESIAN_POINT('Origin',(-45.,-753.32045741381,64.9999999999994));
#131168=CARTESIAN_POINT('Origin',(-55.,366.67954258619,64.9999999999994));
#131169=CARTESIAN_POINT('',(-50.,366.67954258619,72.4999999999994));
#131170=CARTESIAN_POINT('Origin',(-50.,366.67954258619,64.9999999999994));
#131171=CARTESIAN_POINT('',(-45.,366.67954258619,72.4999999999994));
#131172=CARTESIAN_POINT('',(-55.,366.67954258619,72.4999999999994));
#131173=CARTESIAN_POINT('Origin',(-45.,366.67954258619,64.9999999999994));
#131174=CARTESIAN_POINT('Origin',(-55.,-333.32045741381,64.9999999999994));
#131175=CARTESIAN_POINT('',(-50.,-333.32045741381,72.4999999999994));
#131176=CARTESIAN_POINT('Origin',(-50.,-333.32045741381,64.9999999999994));
#131177=CARTESIAN_POINT('',(-45.,-333.32045741381,72.4999999999994));
#131178=CARTESIAN_POINT('',(-55.,-333.32045741381,72.4999999999994));
#131179=CARTESIAN_POINT('Origin',(-45.,-333.32045741381,64.9999999999994));
#131180=CARTESIAN_POINT('Origin',(-55.,86.6795425861912,65.));
#131181=CARTESIAN_POINT('',(-50.,86.6795425861912,72.5));
#131182=CARTESIAN_POINT('Origin',(-50.,86.6795425861912,65.));
#131183=CARTESIAN_POINT('',(-45.,86.6795425861912,72.5));
#131184=CARTESIAN_POINT('',(-55.,86.6795425861912,72.5));
#131185=CARTESIAN_POINT('Origin',(-45.,86.6795425861912,65.));
#131186=CARTESIAN_POINT('Origin',(-55.,786.679542586191,65.));
#131187=CARTESIAN_POINT('',(-50.,786.679542586191,72.5));
#131188=CARTESIAN_POINT('Origin',(-50.,786.679542586191,65.));
#131189=CARTESIAN_POINT('',(-45.,786.679542586191,72.5));
#131190=CARTESIAN_POINT('',(-55.,786.679542586191,72.5));
#131191=CARTESIAN_POINT('Origin',(-45.,786.679542586191,65.));
#131192=CARTESIAN_POINT('Origin',(-55.,646.679542586191,64.9999999999994));
#131193=CARTESIAN_POINT('',(-50.,646.679542586191,72.4999999999994));
#131194=CARTESIAN_POINT('Origin',(-50.,646.679542586191,64.9999999999994));
#131195=CARTESIAN_POINT('',(-45.,646.679542586191,72.4999999999994));
#131196=CARTESIAN_POINT('',(-55.,646.679542586191,72.4999999999994));
#131197=CARTESIAN_POINT('Origin',(-45.,646.679542586191,64.9999999999994));
#131198=CARTESIAN_POINT('Origin',(-55.,506.679542586191,64.9999999999994));
#131199=CARTESIAN_POINT('',(-50.,506.679542586191,72.4999999999994));
#131200=CARTESIAN_POINT('Origin',(-50.,506.679542586191,64.9999999999994));
#131201=CARTESIAN_POINT('',(-45.,506.679542586191,72.4999999999994));
#131202=CARTESIAN_POINT('',(-55.,506.679542586191,72.4999999999994));
#131203=CARTESIAN_POINT('Origin',(-45.,506.679542586191,64.9999999999994));
#131204=CARTESIAN_POINT('Origin',(-55.,226.67954258619,64.9999999999994));
#131205=CARTESIAN_POINT('',(-50.,226.67954258619,72.4999999999994));
#131206=CARTESIAN_POINT('Origin',(-50.,226.67954258619,64.9999999999994));
#131207=CARTESIAN_POINT('',(-45.,226.67954258619,72.4999999999994));
#131208=CARTESIAN_POINT('',(-55.,226.67954258619,72.4999999999994));
#131209=CARTESIAN_POINT('Origin',(-45.,226.67954258619,64.9999999999994));
#131210=CARTESIAN_POINT('Origin',(-55.,-53.3204574138096,64.9999999999994));
#131211=CARTESIAN_POINT('',(-50.,-53.3204574138096,72.4999999999994));
#131212=CARTESIAN_POINT('Origin',(-50.,-53.3204574138096,64.9999999999994));
#131213=CARTESIAN_POINT('',(-45.,-53.3204574138096,72.4999999999994));
#131214=CARTESIAN_POINT('',(-55.,-53.3204574138096,72.4999999999994));
#131215=CARTESIAN_POINT('Origin',(-45.,-53.3204574138096,64.9999999999994));
#131216=CARTESIAN_POINT('Origin',(-55.,-193.32045741381,64.9999999999994));
#131217=CARTESIAN_POINT('',(-50.,-193.32045741381,72.4999999999994));
#131218=CARTESIAN_POINT('Origin',(-50.,-193.32045741381,64.9999999999994));
#131219=CARTESIAN_POINT('',(-45.,-193.32045741381,72.4999999999994));
#131220=CARTESIAN_POINT('',(-55.,-193.32045741381,72.4999999999994));
#131221=CARTESIAN_POINT('Origin',(-45.,-193.32045741381,64.9999999999994));
#131222=CARTESIAN_POINT('Origin',(-55.,-473.32045741381,64.9999999999994));
#131223=CARTESIAN_POINT('',(-50.,-473.32045741381,72.4999999999994));
#131224=CARTESIAN_POINT('Origin',(-50.,-473.32045741381,64.9999999999994));
#131225=CARTESIAN_POINT('',(-45.,-473.32045741381,72.4999999999994));
#131226=CARTESIAN_POINT('',(-55.,-473.32045741381,72.4999999999994));
#131227=CARTESIAN_POINT('Origin',(-45.,-473.32045741381,64.9999999999994));
#131228=CARTESIAN_POINT('Origin',(-55.,-613.32045741381,64.9999999999994));
#131229=CARTESIAN_POINT('',(-50.,-613.32045741381,72.4999999999994));
#131230=CARTESIAN_POINT('Origin',(-50.,-613.32045741381,64.9999999999994));
#131231=CARTESIAN_POINT('',(-45.,-613.32045741381,72.4999999999994));
#131232=CARTESIAN_POINT('',(-55.,-613.32045741381,72.4999999999994));
#131233=CARTESIAN_POINT('Origin',(-45.,-613.32045741381,64.9999999999994));
#131234=CARTESIAN_POINT('Origin',(0.,900.,5.));
#131235=CARTESIAN_POINT('',(0.,-900.,5.));
#131236=CARTESIAN_POINT('',(0.,-900.,0.));
#131237=CARTESIAN_POINT('',(0.,-900.,5.));
#131238=CARTESIAN_POINT('',(0.,900.,0.));
#131239=CARTESIAN_POINT('',(0.,900.,0.));
#131240=CARTESIAN_POINT('',(0.,900.,5.));
#131241=CARTESIAN_POINT('',(0.,900.,5.));
#131242=CARTESIAN_POINT('',(0.,900.,5.));
#131243=CARTESIAN_POINT('Origin',(0.,900.,0.));
#131244=CARTESIAN_POINT('',(-48.,-900.,5.8783046359073E-15));
#131245=CARTESIAN_POINT('',(0.,-900.,0.));
#131246=CARTESIAN_POINT('',(-48.,900.,5.8783046359073E-15));
#131247=CARTESIAN_POINT('',(-48.,900.,5.8783046359073E-15));
#131248=CARTESIAN_POINT('',(0.,900.,0.));
#131249=CARTESIAN_POINT('Origin',(-50.,900.,6.12323399573677E-15));
#131250=CARTESIAN_POINT('',(-50.,-900.,2.00000000000001));
#131251=CARTESIAN_POINT('',(-50.,-900.,128.));
#131252=CARTESIAN_POINT('',(-50.,-900.,6.12323399573677E-15));
#131253=CARTESIAN_POINT('',(-50.,900.,128.));
#131254=CARTESIAN_POINT('',(-50.,900.,128.));
#131255=CARTESIAN_POINT('',(-50.,900.,2.00000000000001));
#131256=CARTESIAN_POINT('',(-50.,900.,6.12323399573677E-15));
#131257=CARTESIAN_POINT('',(-50.,900.,2.00000000000001));
#131258=CARTESIAN_POINT('Origin',(-50.,900.,130.));
#131259=CARTESIAN_POINT('',(-48.,900.,130.));
#131260=CARTESIAN_POINT('',(0.,900.,130.));
#131261=CARTESIAN_POINT('',(-50.,900.,130.));
#131262=CARTESIAN_POINT('',(-48.,-900.,130.));
#131263=CARTESIAN_POINT('',(-48.,900.,130.));
#131264=CARTESIAN_POINT('',(0.,-900.,130.));
#131265=CARTESIAN_POINT('',(-50.,-900.,130.));
#131266=CARTESIAN_POINT('',(0.,900.,130.));
#131267=CARTESIAN_POINT('Origin',(0.,900.,130.));
#131268=CARTESIAN_POINT('',(0.,-900.,125.));
#131269=CARTESIAN_POINT('',(0.,-900.,130.));
#131270=CARTESIAN_POINT('',(0.,900.,125.));
#131271=CARTESIAN_POINT('',(0.,900.,125.));
#131272=CARTESIAN_POINT('',(0.,900.,130.));
#131273=CARTESIAN_POINT('Origin',(0.,900.,125.));
#131274=CARTESIAN_POINT('',(-43.,-900.,125.));
#131275=CARTESIAN_POINT('',(0.,-900.,125.));
#131276=CARTESIAN_POINT('',(-43.,900.,125.));
#131277=CARTESIAN_POINT('',(-43.,900.,125.));
#131278=CARTESIAN_POINT('',(0.,900.,125.));
#131279=CARTESIAN_POINT('Origin',(-45.,900.,125.));
#131280=CARTESIAN_POINT('',(-45.,-900.,123.));
#131281=CARTESIAN_POINT('',(-45.,-900.,7.00000000000001));
#131282=CARTESIAN_POINT('',(-45.,-900.,125.));
#131283=CARTESIAN_POINT('',(-45.,900.,7.00000000000001));
#131284=CARTESIAN_POINT('',(-45.,900.,7.));
#131285=CARTESIAN_POINT('',(-45.,900.,123.));
#131286=CARTESIAN_POINT('',(-45.,900.,125.));
#131287=CARTESIAN_POINT('',(-45.,-900.,123.));
#131288=CARTESIAN_POINT('Origin',(-45.,900.,5.));
#131289=CARTESIAN_POINT('',(-43.,900.,5.));
#131290=CARTESIAN_POINT('',(-45.,900.,5.));
#131291=CARTESIAN_POINT('',(-43.,-900.,5.));
#131292=CARTESIAN_POINT('',(-43.,-900.,5.));
#131293=CARTESIAN_POINT('',(-45.,-900.,5.));
#131294=CARTESIAN_POINT('Origin',(0.,900.,0.));
#131295=CARTESIAN_POINT('Origin',(-48.,900.,128.));
#131296=CARTESIAN_POINT('Origin',(-43.,900.,123.));
#131297=CARTESIAN_POINT('Origin',(-43.,900.,7.));
#131298=CARTESIAN_POINT('Origin',(-48.,900.,2.00000000000001));
#131299=CARTESIAN_POINT('Origin',(0.,-900.,0.));
#131300=CARTESIAN_POINT('Origin',(-48.,-900.,128.));
#131301=CARTESIAN_POINT('Origin',(-48.,-900.,2.00000000000001));
#131302=CARTESIAN_POINT('Origin',(-43.,-900.,7.));
#131303=CARTESIAN_POINT('Origin',(-43.,-900.,123.));
#131304=CARTESIAN_POINT('Origin',(-48.,900.,128.));
#131305=CARTESIAN_POINT('Origin',(-48.,900.,2.00000000000001));
#131306=CARTESIAN_POINT('Origin',(-43.,900.,7.));
#131307=CARTESIAN_POINT('Origin',(-43.,900.,123.));
#310582=UNCERTAINTY_MEASURE_WITH_UNIT(LENGTH_MEASURE(0.01),#310624,
'DISTANCE_ACCURACY_VALUE',
'Maximum model space distance between geometric entities at asserted c
onnectivities');
#310601=UNCERTAINTY_MEASURE_WITH_UNIT(LENGTH_MEASURE(0.01),#310624,
'DISTANCE_ACCURACY_VALUE',
'Maximum model space distance between geometric entities at asserted c
onnectivities');
#310604=(
GEOMETRIC_REPRESENTATION_CONTEXT(3)
GLOBAL_UNCERTAINTY_ASSIGNED_CONTEXT((#310582))
GLOBAL_UNIT_ASSIGNED_CONTEXT((#310624,#310626,#310627))
REPRESENTATION_CONTEXT('','3D')
);
#310623=(
GEOMETRIC_REPRESENTATION_CONTEXT(3)
GLOBAL_UNCERTAINTY_ASSIGNED_CONTEXT((#310601))
GLOBAL_UNIT_ASSIGNED_CONTEXT((#310624,#310626,#310627))
REPRESENTATION_CONTEXT('','3D')
);
#310624=(
LENGTH_UNIT()
NAMED_UNIT(*)
SI_UNIT(.MILLI.,.METRE.)
);
#310626=(
NAMED_UNIT(*)
PLANE_ANGLE_UNIT()
SI_UNIT($,.RADIAN.)
);
#310627=(
NAMED_UNIT(*)
SI_UNIT($,.STERADIAN.)
SOLID_ANGLE_UNIT()
);
#310630=SHAPE_DEFINITION_REPRESENTATION(#310651,#310895);
#310651=PRODUCT_DEFINITION_SHAPE('',$,#310917);
#310895=SHAPE_REPRESENTATION('',(#94023),#310604);
#310914=PRODUCT_DEFINITION_CONTEXT('part definition',#310979,'design');
#310917=PRODUCT_DEFINITION('Left Side Channel Support Rail',
'Left Side Channel Support Rail',#310938,#310914);
#310938=PRODUCT_DEFINITION_FORMATION('',$,#310983);
#310979=APPLICATION_CONTEXT(
'Core Data for Automotive Mechanical Design Process');
#310980=PRODUCT_CONTEXT('part definition',#310979,'mechanical');
#310983=PRODUCT('Left Side Channel Support Rail',
'Left Side Channel Support Rail',$,(#310980));
#311004=PRESENTATION_STYLE_ASSIGNMENT((#311011));
#311011=SURFACE_STYLE_USAGE(.BOTH.,#311018);
#311018=SURFACE_SIDE_STYLE('',(#311025));
#311025=SURFACE_STYLE_FILL_AREA(#311032);
#311032=FILL_AREA_STYLE('Opaque(227,224,212)',(#311039));
#311039=FILL_AREA_STYLE_COLOUR('Opaque(227,224,212)',#311046);
#311046=COLOUR_RGB('Opaque(227,224,212)',0.890196078431372,0.87843137254902,
0.831372549019608);
ENDSEC;
END-ISO-10303-21;
